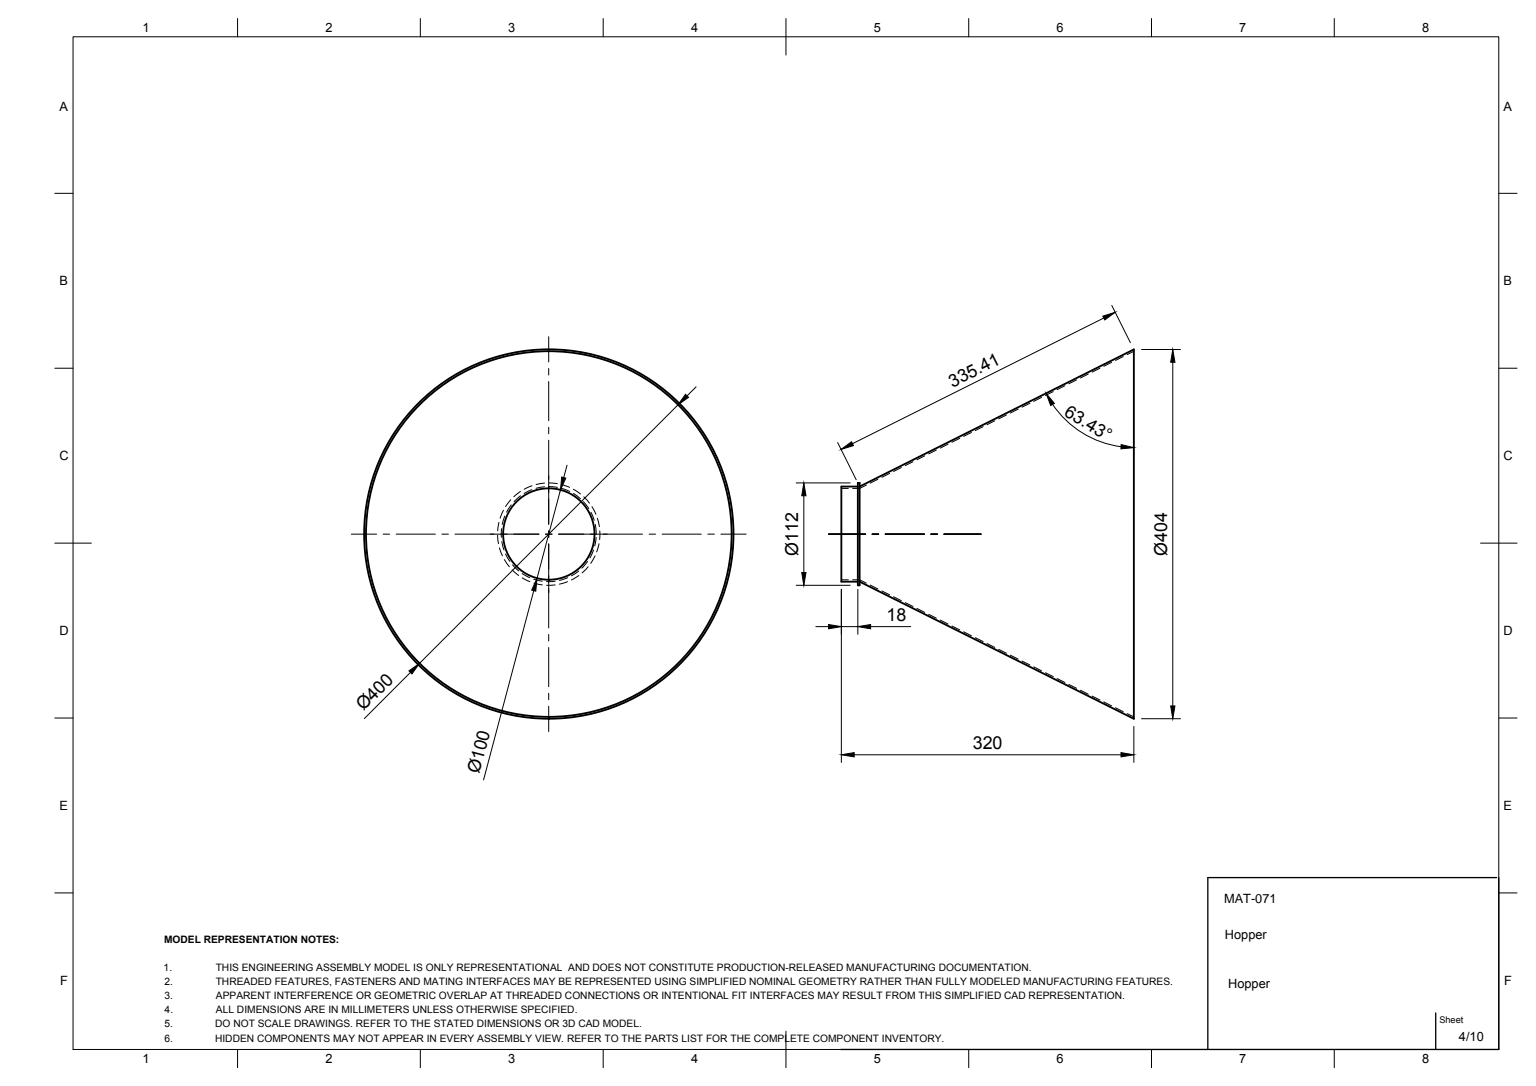
ISO-10303-21;
HEADER;
/* Generated by software containing ST-Developer
 * from STEP Tools, Inc. (www.steptools.com) 
 */

FILE_DESCRIPTION(
/* description */ (''),
/* implementation_level */ '2;1');

FILE_NAME(
/* name */ 'Hopper.step',
/* time_stamp */ '2026-10-24T12:24:47-07:00',
/* author */ (''),
/* organization */ (''),
/* preprocessor_version */ 'ST-DEVELOPER v20.2',
/* originating_system */ 'Autodesk Translation Framework v15.15.0.0',
/* authorisation */ '');

FILE_SCHEMA (('AUTOMOTIVE_DESIGN { 1 0 10303 214 3 1 1 }'));
ENDSEC;

DATA;
#10=MECHANICAL_DESIGN_GEOMETRIC_PRESENTATION_REPRESENTATION('',(#60),#13594);
#48=SHAPE_REPRESENTATION_RELATIONSHIP('SRR','None',#13628,#54);
#54=ADVANCED_BREP_SHAPE_REPRESENTATION('',(#66),#13591);
#60=STYLED_ITEM('',(#13667),#66);
#66=MANIFOLD_SOLID_BREP('Hopper',#2967);
#78=CONICAL_SURFACE('',#3208,52.,0.463647609000806);
#79=CONICAL_SURFACE('',#3210,200.,0.463647609000806);
#95=PLANE('',#3205);
#96=PLANE('',#3217);
#97=PLANE('',#3221);
#98=PLANE('',#3222);
#125=FACE_BOUND('',#525,.T.);
#126=FACE_BOUND('',#531,.T.);
#127=FACE_BOUND('',#534,.T.);
#128=FACE_BOUND('',#536,.T.);
#176=CIRCLE('',#3206,202.);
#177=CIRCLE('',#3207,200.);
#178=CIRCLE('',#3209,52.);
#179=CIRCLE('',#3211,50.);
#180=CIRCLE('',#3213,50.);
#181=CIRCLE('',#3215,52.);
#182=CIRCLE('',#3216,52.);
#183=CIRCLE('',#3219,56.);
#184=CIRCLE('',#3220,56.);
#341=FACE_OUTER_BOUND('',#524,.T.);
#342=FACE_OUTER_BOUND('',#526,.T.);
#343=FACE_OUTER_BOUND('',#527,.T.);
#344=FACE_OUTER_BOUND('',#528,.T.);
#345=FACE_OUTER_BOUND('',#529,.T.);
#346=FACE_OUTER_BOUND('',#530,.T.);
#347=FACE_OUTER_BOUND('',#532,.T.);
#348=FACE_OUTER_BOUND('',#533,.T.);
#349=FACE_OUTER_BOUND('',#535,.T.);
#524=EDGE_LOOP('',(#2527));
#525=EDGE_LOOP('',(#2528));
#526=EDGE_LOOP('',(#2529,#2530,#2531,#2532));
#527=EDGE_LOOP('',(#2533,#2534,#2535,#2536));
#528=EDGE_LOOP('',(#2537,#2538,#2539,#2540));
#529=EDGE_LOOP('',(#2541,#2542,#2543,#2544));
#530=EDGE_LOOP('',(#2545));
#531=EDGE_LOOP('',(#2546));
#532=EDGE_LOOP('',(#2547,#2548,#2549,#2550));
#533=EDGE_LOOP('',(#2551));
#534=EDGE_LOOP('',(#2552));
#535=EDGE_LOOP('',(#2553));
#536=EDGE_LOOP('',(#2554));
#903=LINE('',#11244,#1054);
#904=LINE('',#11249,#1055);
#905=LINE('',#11253,#1056);
#906=LINE('',#11258,#1057);
#907=LINE('',#11265,#1058);
#1054=VECTOR('',#3743,52.);
#1055=VECTOR('',#3750,200.);
#1056=VECTOR('',#3755,50.);
#1057=VECTOR('',#3760,52.);
#1058=VECTOR('',#3769,56.);
#1323=VERTEX_POINT('',#11238);
#1324=VERTEX_POINT('',#11240);
#1325=VERTEX_POINT('',#11243);
#1326=VERTEX_POINT('',#11247);
#1327=VERTEX_POINT('',#11251);
#1328=VERTEX_POINT('',#11255);
#1329=VERTEX_POINT('',#11257);
#1330=VERTEX_POINT('',#11262);
#1331=VERTEX_POINT('',#11264);
#1732=EDGE_CURVE('',#1323,#1323,#176,.T.);
#1733=EDGE_CURVE('',#1324,#1324,#177,.T.);
#1734=EDGE_CURVE('',#1323,#1325,#903,.T.);
#1735=EDGE_CURVE('',#1325,#1325,#178,.T.);
#1736=EDGE_CURVE('',#1326,#1326,#179,.T.);
#1737=EDGE_CURVE('',#1326,#1324,#904,.T.);
#1738=EDGE_CURVE('',#1327,#1327,#180,.F.);
#1739=EDGE_CURVE('',#1327,#1326,#905,.T.);
#1740=EDGE_CURVE('',#1328,#1328,#181,.T.);
#1741=EDGE_CURVE('',#1328,#1329,#906,.T.);
#1742=EDGE_CURVE('',#1329,#1329,#182,.T.);
#1743=EDGE_CURVE('',#1330,#1330,#183,.T.);
#1744=EDGE_CURVE('',#1330,#1331,#907,.T.);
#1745=EDGE_CURVE('',#1331,#1331,#184,.T.);
#2527=ORIENTED_EDGE('',*,*,#1732,.T.);
#2528=ORIENTED_EDGE('',*,*,#1733,.F.);
#2529=ORIENTED_EDGE('',*,*,#1732,.F.);
#2530=ORIENTED_EDGE('',*,*,#1734,.T.);
#2531=ORIENTED_EDGE('',*,*,#1735,.F.);
#2532=ORIENTED_EDGE('',*,*,#1734,.F.);
#2533=ORIENTED_EDGE('',*,*,#1736,.F.);
#2534=ORIENTED_EDGE('',*,*,#1737,.T.);
#2535=ORIENTED_EDGE('',*,*,#1733,.T.);
#2536=ORIENTED_EDGE('',*,*,#1737,.F.);
#2537=ORIENTED_EDGE('',*,*,#1738,.F.);
#2538=ORIENTED_EDGE('',*,*,#1739,.T.);
#2539=ORIENTED_EDGE('',*,*,#1736,.T.);
#2540=ORIENTED_EDGE('',*,*,#1739,.F.);
#2541=ORIENTED_EDGE('',*,*,#1740,.T.);
#2542=ORIENTED_EDGE('',*,*,#1741,.T.);
#2543=ORIENTED_EDGE('',*,*,#1742,.F.);
#2544=ORIENTED_EDGE('',*,*,#1741,.F.);
#2545=ORIENTED_EDGE('',*,*,#1742,.T.);
#2546=ORIENTED_EDGE('',*,*,#1738,.T.);
#2547=ORIENTED_EDGE('',*,*,#1743,.T.);
#2548=ORIENTED_EDGE('',*,*,#1744,.T.);
#2549=ORIENTED_EDGE('',*,*,#1745,.F.);
#2550=ORIENTED_EDGE('',*,*,#1744,.F.);
#2551=ORIENTED_EDGE('',*,*,#1745,.T.);
#2552=ORIENTED_EDGE('',*,*,#1740,.F.);
#2553=ORIENTED_EDGE('',*,*,#1743,.F.);
#2554=ORIENTED_EDGE('',*,*,#1735,.T.);
#2782=CYLINDRICAL_SURFACE('',#3212,50.);
#2783=CYLINDRICAL_SURFACE('',#3214,52.);
#2784=CYLINDRICAL_SURFACE('',#3218,56.);
#2928=ADVANCED_FACE('',(#341,#125),#95,.F.);
#2929=ADVANCED_FACE('',(#342),#78,.T.);
#2930=ADVANCED_FACE('',(#343),#79,.F.);
#2931=ADVANCED_FACE('',(#344),#2782,.F.);
#2932=ADVANCED_FACE('',(#345),#2783,.T.);
#2933=ADVANCED_FACE('',(#346,#126),#96,.T.);
#2934=ADVANCED_FACE('',(#347),#2784,.T.);
#2935=ADVANCED_FACE('',(#348,#127),#97,.T.);
#2936=ADVANCED_FACE('',(#349,#128),#98,.F.);
#2967=CLOSED_SHELL('',(#2928,#2929,#2930,#2931,#2932,#2933,#2934,#2935,
#2936));
#3204=AXIS2_PLACEMENT_3D('',#11236,#3733,#3734);
#3205=AXIS2_PLACEMENT_3D('',#11237,#3735,#3736);
#3206=AXIS2_PLACEMENT_3D('',#11239,#3737,#3738);
#3207=AXIS2_PLACEMENT_3D('',#11241,#3739,#3740);
#3208=AXIS2_PLACEMENT_3D('',#11242,#3741,#3742);
#3209=AXIS2_PLACEMENT_3D('',#11245,#3744,#3745);
#3210=AXIS2_PLACEMENT_3D('',#11246,#3746,#3747);
#3211=AXIS2_PLACEMENT_3D('',#11248,#3748,#3749);
#3212=AXIS2_PLACEMENT_3D('',#11250,#3751,#3752);
#3213=AXIS2_PLACEMENT_3D('',#11252,#3753,#3754);
#3214=AXIS2_PLACEMENT_3D('',#11254,#3756,#3757);
#3215=AXIS2_PLACEMENT_3D('',#11256,#3758,#3759);
#3216=AXIS2_PLACEMENT_3D('',#11259,#3761,#3762);
#3217=AXIS2_PLACEMENT_3D('',#11260,#3763,#3764);
#3218=AXIS2_PLACEMENT_3D('',#11261,#3765,#3766);
#3219=AXIS2_PLACEMENT_3D('',#11263,#3767,#3768);
#3220=AXIS2_PLACEMENT_3D('',#11266,#3770,#3771);
#3221=AXIS2_PLACEMENT_3D('',#11267,#3772,#3773);
#3222=AXIS2_PLACEMENT_3D('',#11268,#3774,#3775);
#3733=DIRECTION('axis',(0.,0.,1.));
#3734=DIRECTION('refdir',(1.,0.,0.));
#3735=DIRECTION('center_axis',(0.,-1.,0.));
#3736=DIRECTION('ref_axis',(0.,0.,-1.));
#3737=DIRECTION('center_axis',(0.,1.,0.));
#3738=DIRECTION('ref_axis',(0.,0.,1.));
#3739=DIRECTION('center_axis',(0.,1.,0.));
#3740=DIRECTION('ref_axis',(0.,0.,1.));
#3741=DIRECTION('center_axis',(0.,1.,0.));
#3742=DIRECTION('ref_axis',(0.,0.,1.));
#3743=DIRECTION('',(5.47678698264202E-17,-0.894427190999916,0.447213595499958));
#3744=DIRECTION('center_axis',(0.,-1.,0.));
#3745=DIRECTION('ref_axis',(0.,0.,-1.));
#3746=DIRECTION('center_axis',(0.,1.,0.));
#3747=DIRECTION('ref_axis',(0.,0.,1.));
#3748=DIRECTION('center_axis',(0.,1.,0.));
#3749=DIRECTION('ref_axis',(0.,0.,1.));
#3750=DIRECTION('',(-5.47678698264202E-17,0.894427190999916,-0.447213595499958));
#3751=DIRECTION('center_axis',(0.,1.,0.));
#3752=DIRECTION('ref_axis',(0.,0.,1.));
#3753=DIRECTION('center_axis',(0.,-1.,0.));
#3754=DIRECTION('ref_axis',(0.,0.,-1.));
#3755=DIRECTION('',(0.,1.,0.));
#3756=DIRECTION('center_axis',(0.,1.,0.));
#3757=DIRECTION('ref_axis',(0.,0.,1.));
#3758=DIRECTION('center_axis',(0.,-1.,0.));
#3759=DIRECTION('ref_axis',(0.,0.,-1.));
#3760=DIRECTION('',(0.,-1.,0.));
#3761=DIRECTION('center_axis',(0.,-1.,0.));
#3762=DIRECTION('ref_axis',(0.,0.,-1.));
#3763=DIRECTION('center_axis',(0.,-1.,0.));
#3764=DIRECTION('ref_axis',(0.,0.,-1.));
#3765=DIRECTION('center_axis',(0.,1.,0.));
#3766=DIRECTION('ref_axis',(0.,0.,1.));
#3767=DIRECTION('center_axis',(0.,-1.,0.));
#3768=DIRECTION('ref_axis',(0.,0.,-1.));
#3769=DIRECTION('',(0.,-1.,0.));
#3770=DIRECTION('center_axis',(0.,-1.,0.));
#3771=DIRECTION('ref_axis',(0.,0.,-1.));
#3772=DIRECTION('center_axis',(0.,-1.,0.));
#3773=DIRECTION('ref_axis',(0.,0.,-1.));
#3774=DIRECTION('center_axis',(0.,-1.,0.));
#3775=DIRECTION('ref_axis',(0.,0.,-1.));
#11236=CARTESIAN_POINT('',(0.,0.,0.));
#11237=CARTESIAN_POINT('Origin',(200.,150.,0.));
#11238=CARTESIAN_POINT('',(-2.47378653427765E-14,150.,-202.));
#11239=CARTESIAN_POINT('Origin',(0.,150.,0.));
#11240=CARTESIAN_POINT('',(-2.44929359829471E-14,150.,-200.));
#11241=CARTESIAN_POINT('Origin',(0.,150.,0.));
#11242=CARTESIAN_POINT('Origin',(0.,-150.,0.));
#11243=CARTESIAN_POINT('',(0.,-150.,-52.));
#11244=CARTESIAN_POINT('',(-6.36816335556624E-15,-150.,-52.));
#11245=CARTESIAN_POINT('Origin',(0.,-150.,0.));
#11246=CARTESIAN_POINT('Origin',(0.,150.,0.));
#11247=CARTESIAN_POINT('',(-6.12323399573677E-15,-150.,-50.0000000000001));
#11248=CARTESIAN_POINT('Origin',(0.,-150.,0.));
#11249=CARTESIAN_POINT('',(-2.44929359829471E-14,150.,-200.));
#11250=CARTESIAN_POINT('Origin',(0.,-170.,0.));
#11251=CARTESIAN_POINT('',(0.,-170.,-50.));
#11252=CARTESIAN_POINT('Origin',(0.,-170.,0.));
#11253=CARTESIAN_POINT('',(-6.12323399573677E-15,-170.,-50.));
#11254=CARTESIAN_POINT('Origin',(0.,-170.,0.));
#11255=CARTESIAN_POINT('',(0.,-152.,-52.));
#11256=CARTESIAN_POINT('Origin',(0.,-152.,0.));
#11257=CARTESIAN_POINT('',(0.,-170.,-52.));
#11258=CARTESIAN_POINT('',(-6.36816335556624E-15,-170.,-52.));
#11259=CARTESIAN_POINT('Origin',(0.,-170.,0.));
#11260=CARTESIAN_POINT('Origin',(0.,-170.,0.));
#11261=CARTESIAN_POINT('Origin',(0.,-152.,0.));
#11262=CARTESIAN_POINT('',(0.,-150.,-56.));
#11263=CARTESIAN_POINT('Origin',(0.,-150.,0.));
#11264=CARTESIAN_POINT('',(0.,-152.,-56.));
#11265=CARTESIAN_POINT('',(-6.85802207522518E-15,-152.,-56.));
#11266=CARTESIAN_POINT('Origin',(0.,-152.,0.));
#11267=CARTESIAN_POINT('Origin',(0.,-152.,0.));
#11268=CARTESIAN_POINT('Origin',(0.,-150.,0.));
#13582=UNCERTAINTY_MEASURE_WITH_UNIT(LENGTH_MEASURE(0.01),#13595,
'DISTANCE_ACCURACY_VALUE',
'Maximum model space distance between geometric entities at asserted c
onnectivities');
#13585=UNCERTAINTY_MEASURE_WITH_UNIT(LENGTH_MEASURE(0.01),#13595,
'DISTANCE_ACCURACY_VALUE',
'Maximum model space distance between geometric entities at asserted c
onnectivities');
#13591=(
GEOMETRIC_REPRESENTATION_CONTEXT(3)
GLOBAL_UNCERTAINTY_ASSIGNED_CONTEXT((#13582))
GLOBAL_UNIT_ASSIGNED_CONTEXT((#13595,#13597,#13598))
REPRESENTATION_CONTEXT('','3D')
);
#13594=(
GEOMETRIC_REPRESENTATION_CONTEXT(3)
GLOBAL_UNCERTAINTY_ASSIGNED_CONTEXT((#13585))
GLOBAL_UNIT_ASSIGNED_CONTEXT((#13595,#13597,#13598))
REPRESENTATION_CONTEXT('','3D')
);
#13595=(
LENGTH_UNIT()
NAMED_UNIT(*)
SI_UNIT(.MILLI.,.METRE.)
);
#13597=(
NAMED_UNIT(*)
PLANE_ANGLE_UNIT()
SI_UNIT($,.RADIAN.)
);
#13598=(
NAMED_UNIT(*)
SI_UNIT($,.STERADIAN.)
SOLID_ANGLE_UNIT()
);
#13604=SHAPE_DEFINITION_REPRESENTATION(#13615,#13628);
#13615=PRODUCT_DEFINITION_SHAPE('',$,#13637);
#13628=SHAPE_REPRESENTATION('',(#3204),#13591);
#13631=PRODUCT_DEFINITION_CONTEXT('part definition',#13657,'design');
#13637=PRODUCT_DEFINITION('Hopper','Hopper',#13645,#13631);
#13645=PRODUCT_DEFINITION_FORMATION('',$,#13664);
#13657=APPLICATION_CONTEXT(
'Core Data for Automotive Mechanical Design Process');
#13658=PRODUCT_CONTEXT('part definition',#13657,'mechanical');
#13664=PRODUCT('Hopper','Hopper',$,(#13658));
#13667=PRESENTATION_STYLE_ASSIGNMENT((#13668));
#13668=SURFACE_STYLE_USAGE(.BOTH.,#13669);
#13669=SURFACE_SIDE_STYLE('',(#13670));
#13670=SURFACE_STYLE_FILL_AREA(#13671);
#13671=FILL_AREA_STYLE('Steel - Satin',(#13672));
#13672=FILL_AREA_STYLE_COLOUR('Steel - Satin',#13673);
#13673=COLOUR_RGB('Steel - Satin',0.627450980392157,0.627450980392157,0.627450980392157);
ENDSEC;
END-ISO-10303-21;
